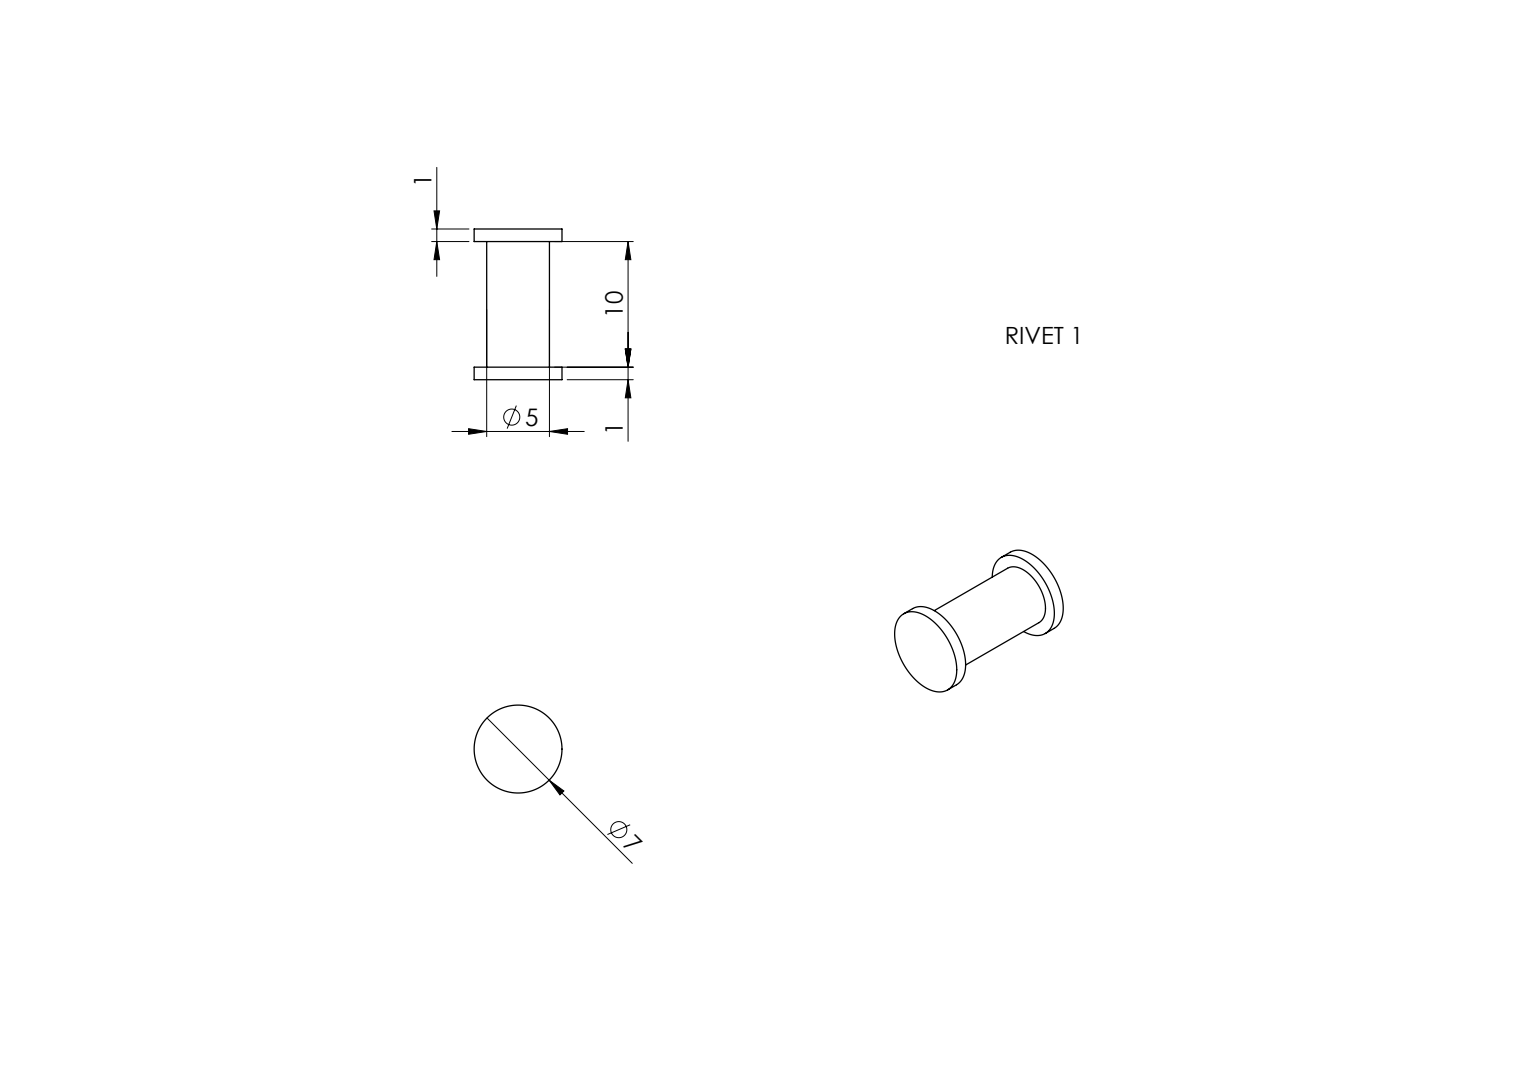
ISO-10303-21;
HEADER;
FILE_DESCRIPTION (('STEP AP214'),
    '1' );
FILE_NAME ('rivet 1.step',
    '2026-10-31T03:36:27',
    ( '' ),
    ( '' ),
    'SwSTEP 2.0',
    'SolidWorks 2026',
    '' );
FILE_SCHEMA (( 'AUTOMOTIVE_DESIGN' ));
ENDSEC;

DATA;
#10=DIRECTION ( 'NONE',  ( 0.000000000000000000, 0.000000000000000000, 1.000000000000000000 ) ) ;
#212=VERTEX_POINT ( 'NONE', #19884 ) ;
#385=DIRECTION ( 'NONE',  ( -1.000000000000000000, 0.000000000000000000, 0.000000000000000000 ) ) ;
#466=DIRECTION ( 'NONE',  ( 0.000000000000000000, 0.000000000000000000, 1.000000000000000000 ) ) ;
#599=ORIENTED_EDGE ( 'NONE', *, *, #8780, .T. ) ;
#763=ORIENTED_EDGE ( 'NONE', *, *, #7373, .F. ) ;
#967=( NAMED_UNIT ( * ) SI_UNIT ( $, .STERADIAN. ) SOLID_ANGLE_UNIT ( ) );
#1179=DIRECTION ( 'NONE',  ( 0.000000000000000000, 0.000000000000000000, 1.000000000000000000 ) ) ;
#1235=DIRECTION ( 'NONE',  ( 1.000000000000000000, 0.000000000000000000, 0.000000000000000000 ) ) ;
#1259=DIRECTION ( 'NONE',  ( -0.000000000000000000, -0.000000000000000000, 1.000000000000000000 ) ) ;
#1401=EDGE_LOOP ( 'NONE', ( #763, #24922, #8044, #21636 ) ) ;
#1450=AXIS2_PLACEMENT_3D ( 'NONE', #34313, #8358, #5492 ) ;
#1710=CLOSED_SHELL ( 'NONE', ( #11763, #6880, #29831, #34272, #5221, #24168, #34342, #28757, #8109, #22910 ) ) ;
#1919=DIRECTION ( 'NONE',  ( -0.000000000000000000, -0.000000000000000000, -1.000000000000000000 ) ) ;
#1930=ORIENTED_EDGE ( 'NONE', *, *, #21548, .F. ) ;
#2055=CARTESIAN_POINT ( 'NONE',  ( 2.999999999999997335, 244.5000000000000000, -10.00000000000000000 ) ) ;
#2478=CARTESIAN_POINT ( 'NONE',  ( -0.5000000000000052180, 244.5000000000000000, -11.00000000000000000 ) ) ;
#2485=CARTESIAN_POINT ( 'NONE',  ( 2.999999999999997335, 244.5000000000000000, 0.000000000000000000 ) ) ;
#2724=AXIS2_PLACEMENT_3D ( 'NONE', #10371, #33121, #18923 ) ;
#2784=CARTESIAN_POINT ( 'NONE',  ( 5.499999999999994671, 244.5000000000000000, 0.000000000000000000 ) ) ;
#2880=PRODUCT ( 'rivet 1', 'rivet 1', '', ( #17586 ) ) ;
#3026=PLANE ( 'NONE',  #24465 ) ;
#3047=ORIENTED_EDGE ( 'NONE', *, *, #8210, .T. ) ;
#3126=EDGE_CURVE ( 'NONE', #32537, #21538, #16483, .T. ) ;
#3249=SURFACE_STYLE_FILL_AREA ( #23539 ) ;
#3629=DIRECTION ( 'NONE',  ( 0.000000000000000000, 0.000000000000000000, 1.000000000000000000 ) ) ;
#3635=AXIS2_PLACEMENT_3D ( 'NONE', #17497, #20911, #5918 ) ;
#3664=EDGE_LOOP ( 'NONE', ( #7038, #31958 ) ) ;
#3742=EDGE_LOOP ( 'NONE', ( #1930, #7681, #28289, #18409 ) ) ;
#3821=ADVANCED_BREP_SHAPE_REPRESENTATION ( '', ( #33058, #17215 ), #19008 ) ;
#4287=AXIS2_PLACEMENT_3D ( 'NONE', #12544, #3629, #18811 ) ;
#4450=CARTESIAN_POINT ( 'NONE',  ( 6.500000000000000000, 244.5000000000000000, 1.000000000000000000 ) ) ;
#4651=DIRECTION ( 'NONE',  ( 0.000000000000000000, 0.000000000000000000, 1.000000000000000000 ) ) ;
#4833=EDGE_CURVE ( 'NONE', #32427, #22420, #23128, .T. ) ;
#5114=CARTESIAN_POINT ( 'NONE',  ( 6.500000000000000888, 244.5000000000000000, -10.00000000000000000 ) ) ;
#5221=ADVANCED_FACE ( 'NONE', ( #22263 ), #24905, .T. ) ;
#5492=DIRECTION ( 'NONE',  ( -1.000000000000000000, 0.000000000000000000, 0.000000000000000000 ) ) ;
#5875=DIRECTION ( 'NONE',  ( -0.000000000000000000, -0.000000000000000000, 1.000000000000000000 ) ) ;
#5918=DIRECTION ( 'NONE',  ( 1.000000000000000000, 0.000000000000000000, 0.000000000000000000 ) ) ;
#6292=CIRCLE ( 'NONE', #23241, 3.500000000000002220 ) ;
#6478=( NAMED_UNIT ( * ) SI_UNIT ( $, .STERADIAN. ) SOLID_ANGLE_UNIT ( ) );
#6581=CIRCLE ( 'NONE', #21722, 2.499999999999996891 ) ;
#6598=UNCERTAINTY_MEASURE_WITH_UNIT (LENGTH_MEASURE( 1.000000000000000082E-05 ), #26556, 'distance_accuracy_value', 'NONE');
#6730=DIRECTION ( 'NONE',  ( 0.000000000000000000, 0.000000000000000000, 1.000000000000000000 ) ) ;
#6880=ADVANCED_FACE ( 'NONE', ( #23612 ), #25708, .T. ) ;
#6896=EDGE_CURVE ( 'NONE', #212, #21530, #20034, .T. ) ;
#7038=ORIENTED_EDGE ( 'NONE', *, *, #12828, .T. ) ;
#7112=CARTESIAN_POINT ( 'NONE',  ( 2.999999999999997335, 244.5000000000000000, -11.00000000000000000 ) ) ;
#7231=ORIENTED_EDGE ( 'NONE', *, *, #12828, .F. ) ;
#7339=DIRECTION ( 'NONE',  ( 1.000000000000000000, 0.000000000000000000, 0.000000000000000000 ) ) ;
#7350=PLANE ( 'NONE',  #2724 ) ;
#7373=EDGE_CURVE ( 'NONE', #32537, #212, #6292, .T. ) ;
#7385=DIRECTION ( 'NONE',  ( -0.000000000000000000, -0.000000000000000000, -1.000000000000000000 ) ) ;
#7681=ORIENTED_EDGE ( 'NONE', *, *, #25380, .F. ) ;
#7920=FACE_OUTER_BOUND ( 'NONE', #36758, .T. ) ;
#7963=VERTEX_POINT ( 'NONE', #31288 ) ;
#8044=ORIENTED_EDGE ( 'NONE', *, *, #16436, .T. ) ;
#8109=ADVANCED_FACE ( 'NONE', ( #37328 ), #3026, .T. ) ;
#8210=EDGE_CURVE ( 'NONE', #30563, #7963, #29282, .T. ) ;
#8283=ORIENTED_EDGE ( 'NONE', *, *, #30986, .T. ) ;
#8358=DIRECTION ( 'NONE',  ( 0.000000000000000000, 0.000000000000000000, -1.000000000000000000 ) ) ;
#8482=CYLINDRICAL_SURFACE ( 'NONE', #35502, 3.500000000000003109 ) ;
#8507=DIRECTION ( 'NONE',  ( -1.000000000000000000, 0.000000000000000000, 0.000000000000000000 ) ) ;
#8552=CARTESIAN_POINT ( 'NONE',  ( 2.999999999999997335, 244.5000000000000000, 0.000000000000000000 ) ) ;
#8648=DIRECTION ( 'NONE',  ( -0.000000000000000000, -0.000000000000000000, -1.000000000000000000 ) ) ;
#8710=COLOUR_RGB ( '',0.8941176470588234615, 0.8941176470588234615, 0.8941176470588234615 ) ;
#8740=FACE_OUTER_BOUND ( 'NONE', #3742, .T. ) ;
#8780=EDGE_CURVE ( 'NONE', #21530, #21538, #11677, .T. ) ;
#8818=CIRCLE ( 'NONE', #26365, 2.499999999999996891 ) ;
#8923=PLANE ( 'NONE',  #22893 ) ;
#9185=DIRECTION ( 'NONE',  ( -1.000000000000000000, 0.000000000000000000, 0.000000000000000000 ) ) ;
#9358=ORIENTED_EDGE ( 'NONE', *, *, #19362, .F. ) ;
#9447=VECTOR ( 'NONE', #1919, 1000.000000000000000 ) ;
#9625=FACE_OUTER_BOUND ( 'NONE', #20074, .T. ) ;
#9698=( LENGTH_UNIT ( ) NAMED_UNIT ( * ) SI_UNIT ( .MILLI., .METRE. ) );
#9756=CIRCLE ( 'NONE', #4287, 3.500000000000002220 ) ;
#10148=EDGE_LOOP ( 'NONE', ( #33076, #37000 ) ) ;
#10211=AXIS2_PLACEMENT_3D ( 'NONE', #33299, #1259, #7339 ) ;
#10313=DIRECTION ( 'NONE',  ( 0.000000000000000000, 0.000000000000000000, -1.000000000000000000 ) ) ;
#10371=CARTESIAN_POINT ( 'NONE',  ( 2.999999999999997335, 244.5000000000000000, 1.000000000000000000 ) ) ;
#10397=SHAPE_REPRESENTATION ( 'rivet 1', ( #17215 ), #19008 ) ;
#10587=DIRECTION ( 'NONE',  ( 1.000000000000000000, 0.000000000000000000, 0.000000000000000000 ) ) ;
#10829=CARTESIAN_POINT ( 'NONE',  ( 6.500000000000000000, 244.5000000000000000, 0.000000000000000000 ) ) ;
#11014=VERTEX_POINT ( 'NONE', #29935 ) ;
#11015=CARTESIAN_POINT ( 'NONE',  ( -0.5000000000000047740, 244.5000000000000000, 0.000000000000000000 ) ) ;
#11121=MECHANICAL_DESIGN_GEOMETRIC_PRESENTATION_REPRESENTATION('',(#16564),#32292);
#11190=DIRECTION ( 'NONE',  ( -1.000000000000000000, 0.000000000000000000, -0.000000000000000000 ) ) ;
#11217=EDGE_CURVE ( 'NONE', #22420, #32427, #6581, .T. ) ;
#11248=VECTOR ( 'NONE', #5875, 1000.000000000000000 ) ;
#11267=ORIENTED_EDGE ( 'NONE', *, *, #26246, .F. ) ;
#11490=DIRECTION ( 'NONE',  ( -0.000000000000000000, -0.000000000000000000, -1.000000000000000000 ) ) ;
#11670=CARTESIAN_POINT ( 'NONE',  ( 2.999999999999997335, 244.5000000000000000, 1.000000000000000000 ) ) ;
#11677=CIRCLE ( 'NONE', #16621, 3.500000000000002220 ) ;
#11763=ADVANCED_FACE ( 'NONE', ( #27417 ), #36132, .T. ) ;
#11766=CYLINDRICAL_SURFACE ( 'NONE', #34372, 2.499999999999997335 ) ;
#12004=ORIENTED_EDGE ( 'NONE', *, *, #11217, .T. ) ;
#12153=( NAMED_UNIT ( * ) PLANE_ANGLE_UNIT ( ) SI_UNIT ( $, .RADIAN. ) );
#12282=PRODUCT_DEFINITION_CONTEXT ( 'detailed design', #17071, 'design' ) ;
#12361=STYLED_ITEM('',(#37528),#33058);
#12544=CARTESIAN_POINT ( 'NONE',  ( 2.999999999999997335, 244.5000000000000000, 0.000000000000000000 ) ) ;
#12601=CARTESIAN_POINT ( 'NONE',  ( 6.500000000000000888, 244.5000000000000000, -11.00000000000000000 ) ) ;
#12729=PRESENTATION_STYLE_ASSIGNMENT (( #29404 ) ) ;
#12828=EDGE_CURVE ( 'NONE', #17773, #34698, #27145, .T. ) ;
#12903=EDGE_CURVE ( 'NONE', #17773, #30563, #24537, .T. ) ;
#12923=ORIENTED_EDGE ( 'NONE', *, *, #12903, .T. ) ;
#13120=LINE ( 'NONE', #36972, #9447 ) ;
#13203=APPLICATION_CONTEXT ( 'automotive_design' ) ;
#13449=DIRECTION ( 'NONE',  ( 0.000000000000000000, 0.000000000000000000, -1.000000000000000000 ) ) ;
#13731=DIRECTION ( 'NONE',  ( -0.000000000000000000, -0.000000000000000000, -1.000000000000000000 ) ) ;
#13932=VECTOR ( 'NONE', #7385, 1000.000000000000000 ) ;
#14243=FACE_BOUND ( 'NONE', #10148, .T. ) ;
#14339=EDGE_CURVE ( 'NONE', #212, #32537, #15762, .T. ) ;
#14682=CARTESIAN_POINT ( 'NONE',  ( 2.999999999999997335, 244.5000000000000000, 0.000000000000000000 ) ) ;
#14764=AXIS2_PLACEMENT_3D ( 'NONE', #30786, #13731, #16389 ) ;
#14997=ORIENTED_EDGE ( 'NONE', *, *, #16436, .F. ) ;
#15029=DIRECTION ( 'NONE',  ( 1.000000000000000000, 0.000000000000000000, 0.000000000000000000 ) ) ;
#15490=ORIENTED_EDGE ( 'NONE', *, *, #12903, .F. ) ;
#15575=( NAMED_UNIT ( * ) PLANE_ANGLE_UNIT ( ) SI_UNIT ( $, .RADIAN. ) );
#15576=CIRCLE ( 'NONE', #30110, 3.500000000000002665 ) ;
#15762=CIRCLE ( 'NONE', #19975, 3.500000000000002220 ) ;
#15835=DIRECTION ( 'NONE',  ( 0.000000000000000000, 0.000000000000000000, 1.000000000000000000 ) ) ;
#15857=AXIS2_PLACEMENT_3D ( 'NONE', #23792, #466, #33069 ) ;
#16047=CARTESIAN_POINT ( 'NONE',  ( 0.000000000000000000, 0.000000000000000000, 0.000000000000000000 ) ) ;
#16295=DIRECTION ( 'NONE',  ( -0.000000000000000000, -0.000000000000000000, -1.000000000000000000 ) ) ;
#16389=DIRECTION ( 'NONE',  ( -1.000000000000000000, 0.000000000000000000, 0.000000000000000000 ) ) ;
#16436=EDGE_CURVE ( 'NONE', #21538, #21530, #9756, .T. ) ;
#16483=LINE ( 'NONE', #21987, #30395 ) ;
#16564=STYLED_ITEM ( 'NONE', ( #12729 ), #3821 ) ;
#16621=AXIS2_PLACEMENT_3D ( 'NONE', #32686, #6730, #36272 ) ;
#17071=APPLICATION_CONTEXT ( 'automotive_design' ) ;
#17205=DIRECTION ( 'NONE',  ( 1.000000000000000000, 0.000000000000000000, 0.000000000000000000 ) ) ;
#17215=AXIS2_PLACEMENT_3D ( 'NONE', #16047, #4651, #19645 ) ;
#17260=CARTESIAN_POINT ( 'NONE',  ( 2.999999999999997335, 244.5000000000000000, -11.00000000000000000 ) ) ;
#17333=ORIENTED_EDGE ( 'NONE', *, *, #4833, .F. ) ;
#17395=DIRECTION ( 'NONE',  ( -0.000000000000000000, -0.000000000000000000, 1.000000000000000000 ) ) ;
#17477=ORIENTED_EDGE ( 'NONE', *, *, #19700, .F. ) ;
#17497=CARTESIAN_POINT ( 'NONE',  ( 2.999999999999997335, 244.5000000000000000, 0.000000000000000000 ) ) ;
#17558=CIRCLE ( 'NONE', #3635, 2.499999999999996891 ) ;
#17586=PRODUCT_CONTEXT ( 'NONE', #13203, 'mechanical' ) ;
#17720=FACE_OUTER_BOUND ( 'NONE', #27952, .T. ) ;
#17773=VERTEX_POINT ( 'NONE', #30053 ) ;
#17902=( LENGTH_UNIT ( ) NAMED_UNIT ( * ) SI_UNIT ( .MILLI., .METRE. ) );
#18064=VECTOR ( 'NONE', #27188, 1000.000000000000000 ) ;
#18212=ORIENTED_EDGE ( 'NONE', *, *, #3126, .F. ) ;
#18367=ORIENTED_EDGE ( 'NONE', *, *, #7373, .T. ) ;
#18409=ORIENTED_EDGE ( 'NONE', *, *, #4833, .T. ) ;
#18429=FILL_AREA_STYLE_COLOUR ( '', #8710 ) ;
#18683=DIRECTION ( 'NONE',  ( -1.000000000000000000, 0.000000000000000000, 0.000000000000000000 ) ) ;
#18706=CARTESIAN_POINT ( 'NONE',  ( 2.999999999999997335, 244.5000000000000000, 0.000000000000000000 ) ) ;
#18749=DIRECTION ( 'NONE',  ( -1.000000000000000000, 0.000000000000000000, -0.000000000000000000 ) ) ;
#18811=DIRECTION ( 'NONE',  ( 1.000000000000000000, 0.000000000000000000, 0.000000000000000000 ) ) ;
#18923=DIRECTION ( 'NONE',  ( 1.000000000000000000, 0.000000000000000000, -0.000000000000000000 ) ) ;
#19008=( GEOMETRIC_REPRESENTATION_CONTEXT ( 3 ) GLOBAL_UNCERTAINTY_ASSIGNED_CONTEXT ( ( #35853 ) ) GLOBAL_UNIT_ASSIGNED_CONTEXT ( ( #9698, #15575, #967 ) ) REPRESENTATION_CONTEXT ( 'NONE', 'WORKASPACE' ) );
#19218=UNCERTAINTY_MEASURE_WITH_UNIT (LENGTH_MEASURE( 1.000000000000000082E-05 ), #17902, 'distance_accuracy_value', 'NONE');
#19242=CIRCLE ( 'NONE', #35557, 3.500000000000002665 ) ;
#19362=EDGE_CURVE ( 'NONE', #11014, #32427, #21796, .T. ) ;
#19645=DIRECTION ( 'NONE',  ( 1.000000000000000000, 0.000000000000000000, 0.000000000000000000 ) ) ;
#19700=EDGE_CURVE ( 'NONE', #28686, #11014, #17558, .T. ) ;
#19884=CARTESIAN_POINT ( 'NONE',  ( -0.5000000000000047740, 244.5000000000000000, 1.000000000000000000 ) ) ;
#19975=AXIS2_PLACEMENT_3D ( 'NONE', #33028, #1179, #15029 ) ;
#20034=LINE ( 'NONE', #28541, #31224 ) ;
#20053=FACE_OUTER_BOUND ( 'NONE', #24464, .T. ) ;
#20074=EDGE_LOOP ( 'NONE', ( #24941, #18367 ) ) ;
#20498=DIRECTION ( 'NONE',  ( 1.000000000000000000, 0.000000000000000000, -0.000000000000000000 ) ) ;
#20845=PRODUCT_DEFINITION_FORMATION_WITH_SPECIFIED_SOURCE ( 'ANY', '', #2880, .NOT_KNOWN. ) ;
#20911=DIRECTION ( 'NONE',  ( 0.000000000000000000, 0.000000000000000000, 1.000000000000000000 ) ) ;
#20948=DIRECTION ( 'NONE',  ( 0.000000000000000000, 0.000000000000000000, -1.000000000000000000 ) ) ;
#21345=DIRECTION ( 'NONE',  ( 1.000000000000000000, 0.000000000000000000, 0.000000000000000000 ) ) ;
#21530=VERTEX_POINT ( 'NONE', #11015 ) ;
#21538=VERTEX_POINT ( 'NONE', #10829 ) ;
#21548=EDGE_CURVE ( 'NONE', #28686, #22420, #13120, .T. ) ;
#21636=ORIENTED_EDGE ( 'NONE', *, *, #6896, .F. ) ;
#21722=AXIS2_PLACEMENT_3D ( 'NONE', #2055, #22724, #10587 ) ;
#21796=LINE ( 'NONE', #33349, #13932 ) ;
#21987=CARTESIAN_POINT ( 'NONE',  ( 6.500000000000000000, 244.5000000000000000, 1.000000000000000000 ) ) ;
#22143=FACE_BOUND ( 'NONE', #32871, .T. ) ;
#22263=FACE_OUTER_BOUND ( 'NONE', #33582, .T. ) ;
#22420=VERTEX_POINT ( 'NONE', #29806 ) ;
#22589=ORIENTED_EDGE ( 'NONE', *, *, #11217, .F. ) ;
#22724=DIRECTION ( 'NONE',  ( 0.000000000000000000, 0.000000000000000000, 1.000000000000000000 ) ) ;
#22893=AXIS2_PLACEMENT_3D ( 'NONE', #2485, #10, #20498 ) ;
#22910=ADVANCED_FACE ( 'NONE', ( #22143, #7920 ), #36522, .F. ) ;
#23128=CIRCLE ( 'NONE', #15857, 2.499999999999996891 ) ;
#23241=AXIS2_PLACEMENT_3D ( 'NONE', #26821, #15835, #21345 ) ;
#23492=AXIS2_PLACEMENT_3D ( 'NONE', #7112, #10313, #18683 ) ;
#23539=FILL_AREA_STYLE ('',( #18429 ) ) ;
#23584=( NAMED_UNIT ( * ) PLANE_ANGLE_UNIT ( ) SI_UNIT ( $, .RADIAN. ) );
#23612=FACE_OUTER_BOUND ( 'NONE', #1401, .T. ) ;
#23792=CARTESIAN_POINT ( 'NONE',  ( 2.999999999999997335, 244.5000000000000000, -10.00000000000000000 ) ) ;
#24168=ADVANCED_FACE ( 'NONE', ( #9625 ), #7350, .T. ) ;
#24268=ORIENTED_EDGE ( 'NONE', *, *, #26246, .T. ) ;
#24424=ORIENTED_EDGE ( 'NONE', *, *, #8780, .F. ) ;
#24464=EDGE_LOOP ( 'NONE', ( #11267, #7231, #12923, #3047 ) ) ;
#24465=AXIS2_PLACEMENT_3D ( 'NONE', #17260, #28801, #11190 ) ;
#24537=LINE ( 'NONE', #12601, #18064 ) ;
#24644=ORIENTED_EDGE ( 'NONE', *, *, #30986, .F. ) ;
#24732=CARTESIAN_POINT ( 'NONE',  ( 0.5000000000000000000, 244.5000000000000000, -10.00000000000000000 ) ) ;
#24852=EDGE_LOOP ( 'NONE', ( #28850, #24268, #8283, #15490 ) ) ;
#24905=CYLINDRICAL_SURFACE ( 'NONE', #14764, 3.500000000000002220 ) ;
#24922=ORIENTED_EDGE ( 'NONE', *, *, #3126, .T. ) ;
#24941=ORIENTED_EDGE ( 'NONE', *, *, #14339, .T. ) ;
#25380=EDGE_CURVE ( 'NONE', #11014, #28686, #8818, .T. ) ;
#25708=CYLINDRICAL_SURFACE ( 'NONE', #33624, 3.500000000000002220 ) ;
#25869=DIRECTION ( 'NONE',  ( -1.000000000000000000, 0.000000000000000000, 0.000000000000000000 ) ) ;
#26155=LINE ( 'NONE', #2478, #11248 ) ;
#26246=EDGE_CURVE ( 'NONE', #34698, #7963, #26155, .T. ) ;
#26365=AXIS2_PLACEMENT_3D ( 'NONE', #18706, #27212, #1235 ) ;
#26556=( LENGTH_UNIT ( ) NAMED_UNIT ( * ) SI_UNIT ( .MILLI., .METRE. ) );
#26745=SURFACE_SIDE_STYLE ('',( #3249 ) ) ;
#26821=CARTESIAN_POINT ( 'NONE',  ( 2.999999999999997335, 244.5000000000000000, 1.000000000000000000 ) ) ;
#27145=CIRCLE ( 'NONE', #23492, 3.500000000000002665 ) ;
#27188=DIRECTION ( 'NONE',  ( -0.000000000000000000, -0.000000000000000000, 1.000000000000000000 ) ) ;
#27212=DIRECTION ( 'NONE',  ( 0.000000000000000000, 0.000000000000000000, 1.000000000000000000 ) ) ;
#27417=FACE_OUTER_BOUND ( 'NONE', #24852, .T. ) ;
#27631=CARTESIAN_POINT ( 'NONE',  ( 2.999999999999997335, 244.5000000000000000, -10.00000000000000000 ) ) ;
#27952=EDGE_LOOP ( 'NONE', ( #17477, #34544, #12004, #9358 ) ) ;
#28041=CARTESIAN_POINT ( 'NONE',  ( -0.5000000000000052180, 244.5000000000000000, -11.00000000000000000 ) ) ;
#28289=ORIENTED_EDGE ( 'NONE', *, *, #19362, .T. ) ;
#28447=FACE_OUTER_BOUND ( 'NONE', #29104, .T. ) ;
#28541=CARTESIAN_POINT ( 'NONE',  ( -0.5000000000000047740, 244.5000000000000000, 1.000000000000000000 ) ) ;
#28686=VERTEX_POINT ( 'NONE', #2784 ) ;
#28697=( GEOMETRIC_REPRESENTATION_CONTEXT ( 3 ) GLOBAL_UNCERTAINTY_ASSIGNED_CONTEXT ( ( #19218 ) ) GLOBAL_UNIT_ASSIGNED_CONTEXT ( ( #17902, #23584, #32289 ) ) REPRESENTATION_CONTEXT ( 'NONE', 'WORKASPACE' ) );
#28707=CYLINDRICAL_SURFACE ( 'NONE', #28865, 2.499999999999997335 ) ;
#28728=DIRECTION ( 'NONE',  ( -1.000000000000000000, 0.000000000000000000, 0.000000000000000000 ) ) ;
#28757=ADVANCED_FACE ( 'NONE', ( #20053 ), #8482, .T. ) ;
#28801=DIRECTION ( 'NONE',  ( 0.000000000000000000, 0.000000000000000000, -1.000000000000000000 ) ) ;
#28850=ORIENTED_EDGE ( 'NONE', *, *, #30011, .F. ) ;
#28865=AXIS2_PLACEMENT_3D ( 'NONE', #14682, #31743, #25869 ) ;
#29104=EDGE_LOOP ( 'NONE', ( #24424, #14997 ) ) ;
#29118=SHAPE_DEFINITION_REPRESENTATION ( #29543, #10397 ) ;
#29282=CIRCLE ( 'NONE', #1450, 3.500000000000002665 ) ;
#29404=SURFACE_STYLE_USAGE ( .BOTH. , #26745 ) ;
#29543=PRODUCT_DEFINITION_SHAPE ( 'NONE', 'NONE',  #32183 ) ;
#29592=SHAPE_REPRESENTATION_RELATIONSHIP ( 'NONE' , 'NONE' ,  #10397, #3821 ) ;
#29806=CARTESIAN_POINT ( 'NONE',  ( 5.499999999999994671, 244.5000000000000000, -10.00000000000000000 ) ) ;
#29831=ADVANCED_FACE ( 'NONE', ( #17720 ), #28707, .T. ) ;
#29935=CARTESIAN_POINT ( 'NONE',  ( 0.5000000000000000000, 244.5000000000000000, 0.000000000000000000 ) ) ;
#30011=EDGE_CURVE ( 'NONE', #34698, #17773, #15576, .T. ) ;
#30053=CARTESIAN_POINT ( 'NONE',  ( 6.500000000000000888, 244.5000000000000000, -11.00000000000000000 ) ) ;
#30110=AXIS2_PLACEMENT_3D ( 'NONE', #35885, #20948, #9185 ) ;
#30395=VECTOR ( 'NONE', #16295, 1000.000000000000000 ) ;
#30563=VERTEX_POINT ( 'NONE', #5114 ) ;
#30786=CARTESIAN_POINT ( 'NONE',  ( 2.999999999999997335, 244.5000000000000000, 1.000000000000000000 ) ) ;
#30986=EDGE_CURVE ( 'NONE', #7963, #30563, #19242, .T. ) ;
#31200=AXIS2_PLACEMENT_3D ( 'NONE', #27631, #36714, #18749 ) ;
#31224=VECTOR ( 'NONE', #8648, 1000.000000000000000 ) ;
#31288=CARTESIAN_POINT ( 'NONE',  ( -0.5000000000000052180, 244.5000000000000000, -10.00000000000000000 ) ) ;
#31743=DIRECTION ( 'NONE',  ( -0.000000000000000000, -0.000000000000000000, -1.000000000000000000 ) ) ;
#31958=ORIENTED_EDGE ( 'NONE', *, *, #30011, .T. ) ;
#31970=CARTESIAN_POINT ( 'NONE',  ( 2.999999999999997335, 244.5000000000000000, -11.00000000000000000 ) ) ;
#32037=DIRECTION ( 'NONE',  ( -0.000000000000000000, -0.000000000000000000, -1.000000000000000000 ) ) ;
#32183=PRODUCT_DEFINITION ( 'UNKNOWN', '', #20845, #12282 ) ;
#32289=( NAMED_UNIT ( * ) SI_UNIT ( $, .STERADIAN. ) SOLID_ANGLE_UNIT ( ) );
#32292=( GEOMETRIC_REPRESENTATION_CONTEXT ( 3 ) GLOBAL_UNCERTAINTY_ASSIGNED_CONTEXT ( ( #6598 ) ) GLOBAL_UNIT_ASSIGNED_CONTEXT ( ( #26556, #12153, #6478 ) ) REPRESENTATION_CONTEXT ( 'NONE', 'WORKASPACE' ) );
#32427=VERTEX_POINT ( 'NONE', #24732 ) ;
#32537=VERTEX_POINT ( 'NONE', #4450 ) ;
#32686=CARTESIAN_POINT ( 'NONE',  ( 2.999999999999997335, 244.5000000000000000, 0.000000000000000000 ) ) ;
#32871=EDGE_LOOP ( 'NONE', ( #17333, #22589 ) ) ;
#32994=ORIENTED_EDGE ( 'NONE', *, *, #8210, .F. ) ;
#33028=CARTESIAN_POINT ( 'NONE',  ( 2.999999999999997335, 244.5000000000000000, 1.000000000000000000 ) ) ;
#33058=MANIFOLD_SOLID_BREP ( 'Boss-Extrude3', #1710 ) ;
#33069=DIRECTION ( 'NONE',  ( 1.000000000000000000, 0.000000000000000000, 0.000000000000000000 ) ) ;
#33076=ORIENTED_EDGE ( 'NONE', *, *, #25380, .T. ) ;
#33121=DIRECTION ( 'NONE',  ( 0.000000000000000000, 0.000000000000000000, 1.000000000000000000 ) ) ;
#33299=CARTESIAN_POINT ( 'NONE',  ( 2.999999999999997335, 244.5000000000000000, -11.00000000000000000 ) ) ;
#33349=CARTESIAN_POINT ( 'NONE',  ( 0.5000000000000000000, 244.5000000000000000, 0.000000000000000000 ) ) ;
#33558=MECHANICAL_DESIGN_GEOMETRIC_PRESENTATION_REPRESENTATION('',(#12361),#28697);
#33582=EDGE_LOOP ( 'NONE', ( #18212, #34377, #33642, #599 ) ) ;
#33624=AXIS2_PLACEMENT_3D ( 'NONE', #11670, #11490, #28728 ) ;
#33642=ORIENTED_EDGE ( 'NONE', *, *, #6896, .T. ) ;
#34272=ADVANCED_FACE ( 'NONE', ( #8740 ), #11766, .T. ) ;
#34313=CARTESIAN_POINT ( 'NONE',  ( 2.999999999999997335, 244.5000000000000000, -10.00000000000000000 ) ) ;
#34342=ADVANCED_FACE ( 'NONE', ( #14243, #28447 ), #8923, .F. ) ;
#34372=AXIS2_PLACEMENT_3D ( 'NONE', #8552, #32037, #385 ) ;
#34377=ORIENTED_EDGE ( 'NONE', *, *, #14339, .F. ) ;
#34464=CARTESIAN_POINT ( 'NONE',  ( 2.999999999999997335, 244.5000000000000000, -10.00000000000000000 ) ) ;
#34544=ORIENTED_EDGE ( 'NONE', *, *, #21548, .T. ) ;
#34698=VERTEX_POINT ( 'NONE', #28041 ) ;
#35502=AXIS2_PLACEMENT_3D ( 'NONE', #31970, #17395, #17205 ) ;
#35557=AXIS2_PLACEMENT_3D ( 'NONE', #34464, #13449, #8507 ) ;
#35853=UNCERTAINTY_MEASURE_WITH_UNIT (LENGTH_MEASURE( 1.000000000000000082E-05 ), #9698, 'distance_accuracy_value', 'NONE');
#35885=CARTESIAN_POINT ( 'NONE',  ( 2.999999999999997335, 244.5000000000000000, -11.00000000000000000 ) ) ;
#36132=CYLINDRICAL_SURFACE ( 'NONE', #10211, 3.500000000000003109 ) ;
#36272=DIRECTION ( 'NONE',  ( 1.000000000000000000, 0.000000000000000000, 0.000000000000000000 ) ) ;
#36522=PLANE ( 'NONE',  #31200 ) ;
#36714=DIRECTION ( 'NONE',  ( 0.000000000000000000, 0.000000000000000000, -1.000000000000000000 ) ) ;
#36758=EDGE_LOOP ( 'NONE', ( #32994, #24644 ) ) ;
#36972=CARTESIAN_POINT ( 'NONE',  ( 5.499999999999994671, 244.5000000000000000, 0.000000000000000000 ) ) ;
#37000=ORIENTED_EDGE ( 'NONE', *, *, #19700, .T. ) ;
#37328=FACE_OUTER_BOUND ( 'NONE', #3664, .T. ) ;
#37522=COLOUR_RGB('Light Blue',0.38,0.62,0.78);
#37523=FILL_AREA_STYLE_COLOUR('',#37522);
#37524=FILL_AREA_STYLE('',(#37523));
#37525=SURFACE_STYLE_FILL_AREA(#37524);
#37526=SURFACE_SIDE_STYLE('',(#37525));
#37527=SURFACE_STYLE_USAGE(.BOTH.,#37526);
#37528=PRESENTATION_STYLE_ASSIGNMENT((#37527));
ENDSEC;
END-ISO-10303-21;
